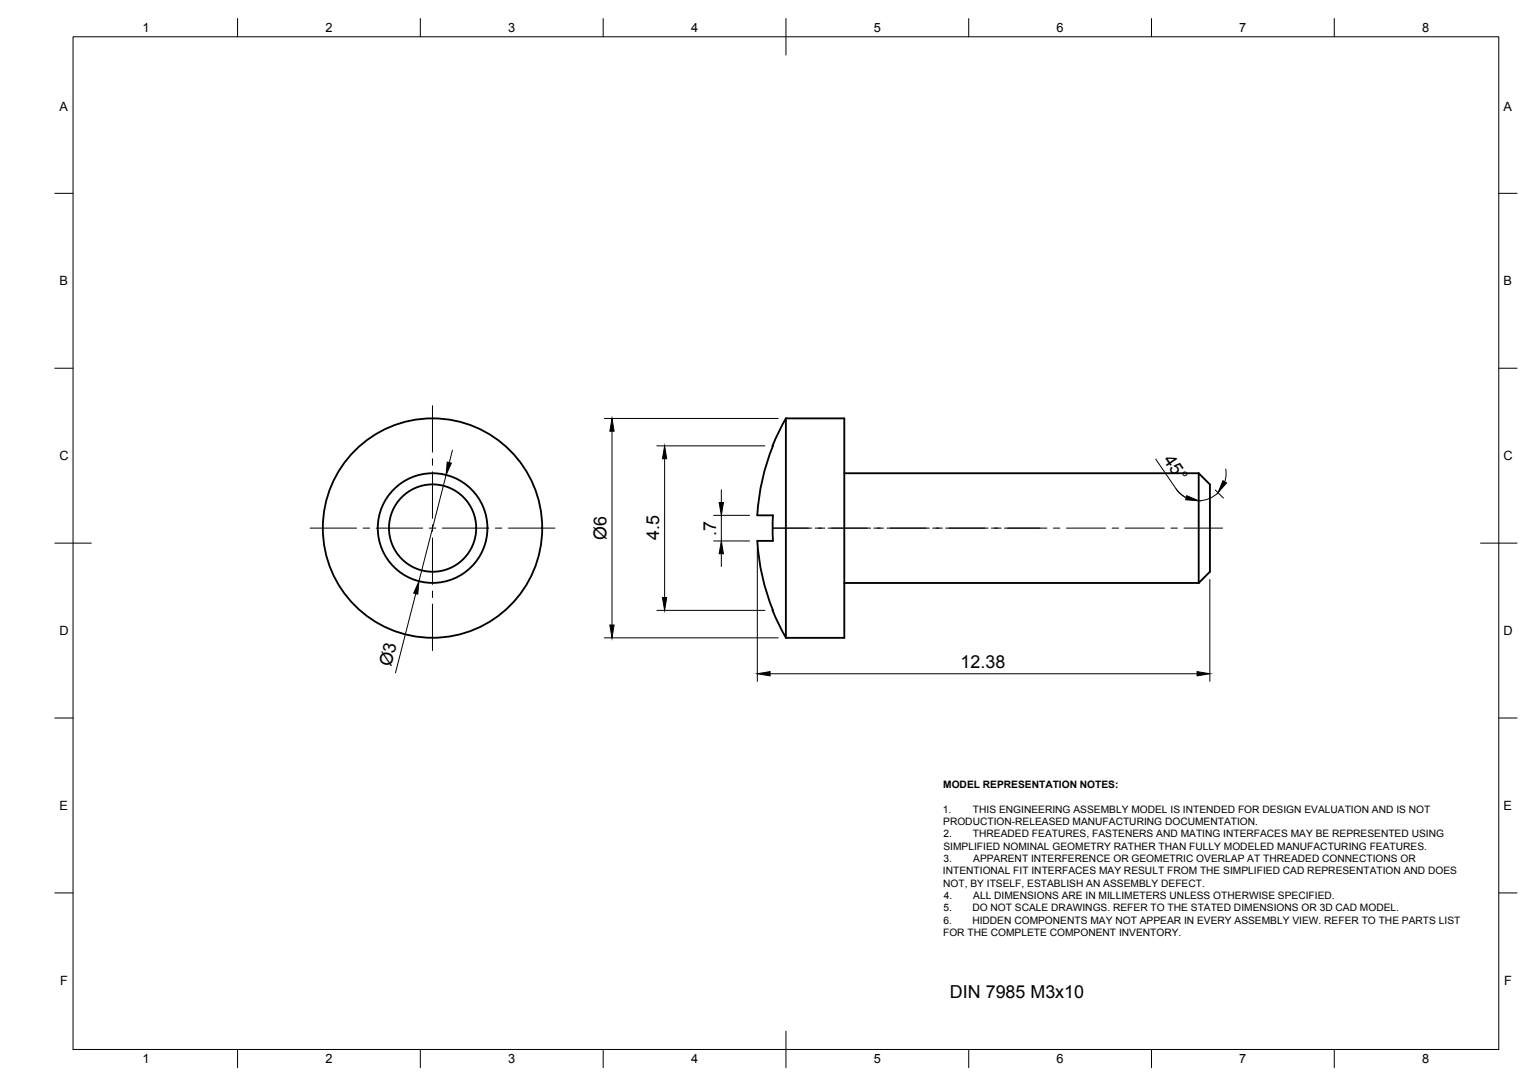
ISO-10303-21;
HEADER;
/* Generated by software containing ST-Developer
 * from STEP Tools, Inc. (www.steptools.com) 
 */

FILE_DESCRIPTION(
/* description */ ('STEP AP214'),
/* implementation_level */ '2;1');

FILE_NAME(
/* name */ 'DIN 7985 M3x10.step',
/* time_stamp */ '2026-10-07T12:18:07-07:00',
/* author */ (''),
/* organization */ (''),
/* preprocessor_version */ 'ST-DEVELOPER v20.2',
/* originating_system */ 'Autodesk Translation Framework v15.15.0.0',
/* authorisation */ '');

FILE_SCHEMA (('AUTOMOTIVE_DESIGN { 1 0 10303 214 3 1 1 }'));
ENDSEC;

DATA;
#10=MECHANICAL_DESIGN_GEOMETRIC_PRESENTATION_REPRESENTATION('',(#127),#62974);
#82=SPHERICAL_SURFACE('',#16177,6.);
#103=SHAPE_REPRESENTATION_RELATIONSHIP('SRR','None',#63026,#115);
#115=ADVANCED_BREP_SHAPE_REPRESENTATION('',(#139),#62967);
#127=STYLED_ITEM('',(#63090),#139);
#139=MANIFOLD_SOLID_BREP('Body1',#15197);
#232=FACE_BOUND('',#5073,.T.);
#233=FACE_BOUND('',#5078,.T.);
#574=PLANE('',#16199);
#575=PLANE('',#16200);
#576=PLANE('',#16201);
#577=PLANE('',#16202);
#578=PLANE('',#16203);
#579=PLANE('',#16204);
#580=PLANE('',#16205);
#581=PLANE('',#16206);
#582=PLANE('',#16207);
#583=PLANE('',#16208);
#584=PLANE('',#16209);
#585=PLANE('',#16210);
#586=PLANE('',#16211);
#587=PLANE('',#16212);
#588=PLANE('',#16213);
#1042=CONICAL_SURFACE('',#16191,1.1935,0.785398163397446);
#1776=LINE('',#44469,#2969);
#1777=LINE('',#44474,#2970);
#1778=LINE('',#44479,#2971);
#1779=LINE('',#44483,#2972);
#1780=LINE('',#44485,#2973);
#1781=LINE('',#44486,#2974);
#1782=LINE('',#44489,#2975);
#1783=LINE('',#44490,#2976);
#1784=LINE('',#44493,#2977);
#1785=LINE('',#44494,#2978);
#1786=LINE('',#44497,#2979);
#1787=LINE('',#44498,#2980);
#1788=LINE('',#44501,#2981);
#1789=LINE('',#44502,#2982);
#1790=LINE('',#44505,#2983);
#1791=LINE('',#44506,#2984);
#1792=LINE('',#44509,#2985);
#1793=LINE('',#44510,#2986);
#1794=LINE('',#44513,#2987);
#1795=LINE('',#44514,#2988);
#1796=LINE('',#44517,#2989);
#1797=LINE('',#44518,#2990);
#1798=LINE('',#44521,#2991);
#1799=LINE('',#44522,#2992);
#1800=LINE('',#44525,#2993);
#1801=LINE('',#44526,#2994);
#1802=LINE('',#44528,#2995);
#2969=VECTOR('',#19387,1.1935);
#2970=VECTOR('',#19394,3.);
#2971=VECTOR('',#19401,1.5);
#2972=VECTOR('',#19406,1000.);
#2973=VECTOR('',#19407,1000.);
#2974=VECTOR('',#19408,1000.);
#2975=VECTOR('',#19411,1000.);
#2976=VECTOR('',#19412,1000.);
#2977=VECTOR('',#19415,1000.);
#2978=VECTOR('',#19416,1000.);
#2979=VECTOR('',#19419,1000.);
#2980=VECTOR('',#19420,1000.);
#2981=VECTOR('',#19423,1000.);
#2982=VECTOR('',#19424,1000.);
#2983=VECTOR('',#19427,1000.);
#2984=VECTOR('',#19428,1000.);
#2985=VECTOR('',#19431,1000.);
#2986=VECTOR('',#19432,1000.);
#2987=VECTOR('',#19435,1000.);
#2988=VECTOR('',#19436,1000.);
#2989=VECTOR('',#19439,1000.);
#2990=VECTOR('',#19440,1000.);
#2991=VECTOR('',#19443,1000.);
#2992=VECTOR('',#19444,1000.);
#2993=VECTOR('',#19447,1000.);
#2994=VECTOR('',#19448,1000.);
#2995=VECTOR('',#19451,1000.);
#3545=CYLINDRICAL_SURFACE('',#16195,3.);
#3546=CYLINDRICAL_SURFACE('',#16197,1.5);
#4167=FACE_OUTER_BOUND('',#5072,.T.);
#4168=FACE_OUTER_BOUND('',#5074,.T.);
#4169=FACE_OUTER_BOUND('',#5075,.T.);
#4170=FACE_OUTER_BOUND('',#5076,.T.);
#4171=FACE_OUTER_BOUND('',#5077,.T.);
#4172=FACE_OUTER_BOUND('',#5079,.T.);
#4173=FACE_OUTER_BOUND('',#5080,.T.);
#4174=FACE_OUTER_BOUND('',#5081,.T.);
#4175=FACE_OUTER_BOUND('',#5082,.T.);
#4176=FACE_OUTER_BOUND('',#5083,.T.);
#4177=FACE_OUTER_BOUND('',#5084,.T.);
#4178=FACE_OUTER_BOUND('',#5085,.T.);
#4179=FACE_OUTER_BOUND('',#5086,.T.);
#4180=FACE_OUTER_BOUND('',#5087,.T.);
#4181=FACE_OUTER_BOUND('',#5088,.T.);
#4182=FACE_OUTER_BOUND('',#5089,.T.);
#4183=FACE_OUTER_BOUND('',#5090,.T.);
#4184=FACE_OUTER_BOUND('',#5091,.T.);
#4185=FACE_OUTER_BOUND('',#5092,.T.);
#5072=EDGE_LOOP('',(#12237));
#5073=EDGE_LOOP('',(#12238,#12239,#12240,#12241,#12242,#12243,#12244,#12245,
#12246,#12247,#12248,#12249));
#5074=EDGE_LOOP('',(#12250,#12251,#12252,#12253,#12254));
#5075=EDGE_LOOP('',(#12255,#12256,#12257,#12258));
#5076=EDGE_LOOP('',(#12259,#12260,#12261,#12262,#12263));
#5077=EDGE_LOOP('',(#12264));
#5078=EDGE_LOOP('',(#12265));
#5079=EDGE_LOOP('',(#12266,#12267,#12268,#12269));
#5080=EDGE_LOOP('',(#12270,#12271,#12272,#12273));
#5081=EDGE_LOOP('',(#12274,#12275,#12276,#12277));
#5082=EDGE_LOOP('',(#12278,#12279,#12280,#12281));
#5083=EDGE_LOOP('',(#12282,#12283,#12284,#12285));
#5084=EDGE_LOOP('',(#12286,#12287,#12288,#12289));
#5085=EDGE_LOOP('',(#12290,#12291,#12292,#12293));
#5086=EDGE_LOOP('',(#12294,#12295,#12296,#12297));
#5087=EDGE_LOOP('',(#12298,#12299,#12300,#12301));
#5088=EDGE_LOOP('',(#12302,#12303,#12304,#12305));
#5089=EDGE_LOOP('',(#12306,#12307,#12308,#12309));
#5090=EDGE_LOOP('',(#12310,#12311,#12312,#12313));
#5091=EDGE_LOOP('',(#12314,#12315,#12316,#12317,#12318,#12319,#12320,#12321,
#12322,#12323,#12324,#12325));
#5092=EDGE_LOOP('',(#12326));
#5854=CIRCLE('',#16178,3.);
#5855=CIRCLE('',#16179,5.56214886532177);
#5856=CIRCLE('',#16180,5.9897829676876);
#5857=CIRCLE('',#16181,5.9897829676876);
#5858=CIRCLE('',#16182,5.5621488653218);
#5859=CIRCLE('',#16183,5.98978296768761);
#5860=CIRCLE('',#16184,5.9897829676876);
#5861=CIRCLE('',#16185,5.56214886532182);
#5862=CIRCLE('',#16186,5.9897829676876);
#5863=CIRCLE('',#16187,5.98978296768761);
#5864=CIRCLE('',#16188,5.5621488653218);
#5865=CIRCLE('',#16189,5.9897829676876);
#5866=CIRCLE('',#16190,5.9897829676876);
#5867=CIRCLE('',#16192,1.5);
#5868=CIRCLE('',#16193,1.1935);
#5869=CIRCLE('',#16194,1.5);
#5870=CIRCLE('',#16196,3.);
#5871=CIRCLE('',#16198,1.5);
#6980=VERTEX_POINT('',#44438);
#6981=VERTEX_POINT('',#44440);
#6982=VERTEX_POINT('',#44441);
#6983=VERTEX_POINT('',#44443);
#6984=VERTEX_POINT('',#44445);
#6985=VERTEX_POINT('',#44447);
#6986=VERTEX_POINT('',#44449);
#6987=VERTEX_POINT('',#44451);
#6988=VERTEX_POINT('',#44453);
#6989=VERTEX_POINT('',#44455);
#6990=VERTEX_POINT('',#44457);
#6991=VERTEX_POINT('',#44459);
#6992=VERTEX_POINT('',#44461);
#6993=VERTEX_POINT('',#44465);
#6994=VERTEX_POINT('',#44466);
#6995=VERTEX_POINT('',#44468);
#6996=VERTEX_POINT('',#44473);
#6997=VERTEX_POINT('',#44477);
#6998=VERTEX_POINT('',#44482);
#6999=VERTEX_POINT('',#44484);
#7000=VERTEX_POINT('',#44488);
#7001=VERTEX_POINT('',#44492);
#7002=VERTEX_POINT('',#44496);
#7003=VERTEX_POINT('',#44500);
#7004=VERTEX_POINT('',#44504);
#7005=VERTEX_POINT('',#44508);
#7006=VERTEX_POINT('',#44512);
#7007=VERTEX_POINT('',#44516);
#7008=VERTEX_POINT('',#44520);
#7009=VERTEX_POINT('',#44524);
#8825=EDGE_CURVE('',#6980,#6980,#5854,.T.);
#8826=EDGE_CURVE('',#6981,#6982,#5855,.T.);
#8827=EDGE_CURVE('',#6982,#6983,#5856,.T.);
#8828=EDGE_CURVE('',#6983,#6984,#5857,.T.);
#8829=EDGE_CURVE('',#6984,#6985,#5858,.T.);
#8830=EDGE_CURVE('',#6985,#6986,#5859,.T.);
#8831=EDGE_CURVE('',#6986,#6987,#5860,.T.);
#8832=EDGE_CURVE('',#6987,#6988,#5861,.T.);
#8833=EDGE_CURVE('',#6988,#6989,#5862,.T.);
#8834=EDGE_CURVE('',#6989,#6990,#5863,.T.);
#8835=EDGE_CURVE('',#6990,#6991,#5864,.T.);
#8836=EDGE_CURVE('',#6991,#6992,#5865,.T.);
#8837=EDGE_CURVE('',#6992,#6981,#5866,.T.);
#8838=EDGE_CURVE('',#6993,#6994,#5867,.T.);
#8839=EDGE_CURVE('',#6994,#6995,#1776,.T.);
#8840=EDGE_CURVE('',#6995,#6995,#5868,.T.);
#8841=EDGE_CURVE('',#6994,#6993,#5869,.T.);
#8842=EDGE_CURVE('',#6980,#6996,#1777,.T.);
#8843=EDGE_CURVE('',#6996,#6996,#5870,.T.);
#8844=EDGE_CURVE('',#6997,#6997,#5871,.T.);
#8845=EDGE_CURVE('',#6997,#6993,#1778,.T.);
#8846=EDGE_CURVE('',#6998,#6991,#1779,.T.);
#8847=EDGE_CURVE('',#6998,#6999,#1780,.T.);
#8848=EDGE_CURVE('',#6999,#6992,#1781,.T.);
#8849=EDGE_CURVE('',#6999,#7000,#1782,.T.);
#8850=EDGE_CURVE('',#7000,#6981,#1783,.T.);
#8851=EDGE_CURVE('',#7000,#7001,#1784,.T.);
#8852=EDGE_CURVE('',#7001,#6982,#1785,.T.);
#8853=EDGE_CURVE('',#7001,#7002,#1786,.T.);
#8854=EDGE_CURVE('',#7002,#6983,#1787,.T.);
#8855=EDGE_CURVE('',#7002,#7003,#1788,.T.);
#8856=EDGE_CURVE('',#7003,#6984,#1789,.T.);
#8857=EDGE_CURVE('',#7003,#7004,#1790,.T.);
#8858=EDGE_CURVE('',#7004,#6985,#1791,.T.);
#8859=EDGE_CURVE('',#7005,#6990,#1792,.T.);
#8860=EDGE_CURVE('',#7005,#6998,#1793,.T.);
#8861=EDGE_CURVE('',#7006,#6989,#1794,.T.);
#8862=EDGE_CURVE('',#7006,#7005,#1795,.T.);
#8863=EDGE_CURVE('',#7004,#7007,#1796,.T.);
#8864=EDGE_CURVE('',#7007,#6986,#1797,.T.);
#8865=EDGE_CURVE('',#7007,#7008,#1798,.T.);
#8866=EDGE_CURVE('',#7008,#6987,#1799,.T.);
#8867=EDGE_CURVE('',#7009,#6988,#1800,.T.);
#8868=EDGE_CURVE('',#7009,#7006,#1801,.T.);
#8869=EDGE_CURVE('',#7008,#7009,#1802,.T.);
#12237=ORIENTED_EDGE('',*,*,#8825,.F.);
#12238=ORIENTED_EDGE('',*,*,#8826,.T.);
#12239=ORIENTED_EDGE('',*,*,#8827,.T.);
#12240=ORIENTED_EDGE('',*,*,#8828,.T.);
#12241=ORIENTED_EDGE('',*,*,#8829,.T.);
#12242=ORIENTED_EDGE('',*,*,#8830,.T.);
#12243=ORIENTED_EDGE('',*,*,#8831,.T.);
#12244=ORIENTED_EDGE('',*,*,#8832,.T.);
#12245=ORIENTED_EDGE('',*,*,#8833,.T.);
#12246=ORIENTED_EDGE('',*,*,#8834,.T.);
#12247=ORIENTED_EDGE('',*,*,#8835,.T.);
#12248=ORIENTED_EDGE('',*,*,#8836,.T.);
#12249=ORIENTED_EDGE('',*,*,#8837,.T.);
#12250=ORIENTED_EDGE('',*,*,#8838,.T.);
#12251=ORIENTED_EDGE('',*,*,#8839,.T.);
#12252=ORIENTED_EDGE('',*,*,#8840,.F.);
#12253=ORIENTED_EDGE('',*,*,#8839,.F.);
#12254=ORIENTED_EDGE('',*,*,#8841,.T.);
#12255=ORIENTED_EDGE('',*,*,#8825,.T.);
#12256=ORIENTED_EDGE('',*,*,#8842,.T.);
#12257=ORIENTED_EDGE('',*,*,#8843,.F.);
#12258=ORIENTED_EDGE('',*,*,#8842,.F.);
#12259=ORIENTED_EDGE('',*,*,#8844,.T.);
#12260=ORIENTED_EDGE('',*,*,#8845,.T.);
#12261=ORIENTED_EDGE('',*,*,#8841,.F.);
#12262=ORIENTED_EDGE('',*,*,#8838,.F.);
#12263=ORIENTED_EDGE('',*,*,#8845,.F.);
#12264=ORIENTED_EDGE('',*,*,#8843,.T.);
#12265=ORIENTED_EDGE('',*,*,#8844,.F.);
#12266=ORIENTED_EDGE('',*,*,#8846,.F.);
#12267=ORIENTED_EDGE('',*,*,#8847,.T.);
#12268=ORIENTED_EDGE('',*,*,#8848,.T.);
#12269=ORIENTED_EDGE('',*,*,#8836,.F.);
#12270=ORIENTED_EDGE('',*,*,#8848,.F.);
#12271=ORIENTED_EDGE('',*,*,#8849,.T.);
#12272=ORIENTED_EDGE('',*,*,#8850,.T.);
#12273=ORIENTED_EDGE('',*,*,#8837,.F.);
#12274=ORIENTED_EDGE('',*,*,#8850,.F.);
#12275=ORIENTED_EDGE('',*,*,#8851,.T.);
#12276=ORIENTED_EDGE('',*,*,#8852,.T.);
#12277=ORIENTED_EDGE('',*,*,#8826,.F.);
#12278=ORIENTED_EDGE('',*,*,#8852,.F.);
#12279=ORIENTED_EDGE('',*,*,#8853,.T.);
#12280=ORIENTED_EDGE('',*,*,#8854,.T.);
#12281=ORIENTED_EDGE('',*,*,#8827,.F.);
#12282=ORIENTED_EDGE('',*,*,#8854,.F.);
#12283=ORIENTED_EDGE('',*,*,#8855,.T.);
#12284=ORIENTED_EDGE('',*,*,#8856,.T.);
#12285=ORIENTED_EDGE('',*,*,#8828,.F.);
#12286=ORIENTED_EDGE('',*,*,#8856,.F.);
#12287=ORIENTED_EDGE('',*,*,#8857,.T.);
#12288=ORIENTED_EDGE('',*,*,#8858,.T.);
#12289=ORIENTED_EDGE('',*,*,#8829,.F.);
#12290=ORIENTED_EDGE('',*,*,#8859,.F.);
#12291=ORIENTED_EDGE('',*,*,#8860,.T.);
#12292=ORIENTED_EDGE('',*,*,#8846,.T.);
#12293=ORIENTED_EDGE('',*,*,#8835,.F.);
#12294=ORIENTED_EDGE('',*,*,#8861,.F.);
#12295=ORIENTED_EDGE('',*,*,#8862,.T.);
#12296=ORIENTED_EDGE('',*,*,#8859,.T.);
#12297=ORIENTED_EDGE('',*,*,#8834,.F.);
#12298=ORIENTED_EDGE('',*,*,#8858,.F.);
#12299=ORIENTED_EDGE('',*,*,#8863,.T.);
#12300=ORIENTED_EDGE('',*,*,#8864,.T.);
#12301=ORIENTED_EDGE('',*,*,#8830,.F.);
#12302=ORIENTED_EDGE('',*,*,#8864,.F.);
#12303=ORIENTED_EDGE('',*,*,#8865,.T.);
#12304=ORIENTED_EDGE('',*,*,#8866,.T.);
#12305=ORIENTED_EDGE('',*,*,#8831,.F.);
#12306=ORIENTED_EDGE('',*,*,#8867,.F.);
#12307=ORIENTED_EDGE('',*,*,#8868,.T.);
#12308=ORIENTED_EDGE('',*,*,#8861,.T.);
#12309=ORIENTED_EDGE('',*,*,#8833,.F.);
#12310=ORIENTED_EDGE('',*,*,#8866,.F.);
#12311=ORIENTED_EDGE('',*,*,#8869,.T.);
#12312=ORIENTED_EDGE('',*,*,#8867,.T.);
#12313=ORIENTED_EDGE('',*,*,#8832,.F.);
#12314=ORIENTED_EDGE('',*,*,#8869,.F.);
#12315=ORIENTED_EDGE('',*,*,#8865,.F.);
#12316=ORIENTED_EDGE('',*,*,#8863,.F.);
#12317=ORIENTED_EDGE('',*,*,#8857,.F.);
#12318=ORIENTED_EDGE('',*,*,#8855,.F.);
#12319=ORIENTED_EDGE('',*,*,#8853,.F.);
#12320=ORIENTED_EDGE('',*,*,#8851,.F.);
#12321=ORIENTED_EDGE('',*,*,#8849,.F.);
#12322=ORIENTED_EDGE('',*,*,#8847,.F.);
#12323=ORIENTED_EDGE('',*,*,#8860,.F.);
#12324=ORIENTED_EDGE('',*,*,#8862,.F.);
#12325=ORIENTED_EDGE('',*,*,#8868,.F.);
#12326=ORIENTED_EDGE('',*,*,#8840,.T.);
#14802=ADVANCED_FACE('',(#4167,#232),#82,.T.);
#14803=ADVANCED_FACE('',(#4168),#1042,.T.);
#14804=ADVANCED_FACE('',(#4169),#3545,.T.);
#14805=ADVANCED_FACE('',(#4170),#3546,.T.);
#14806=ADVANCED_FACE('',(#4171,#233),#574,.T.);
#14807=ADVANCED_FACE('',(#4172),#575,.T.);
#14808=ADVANCED_FACE('',(#4173),#576,.T.);
#14809=ADVANCED_FACE('',(#4174),#577,.T.);
#14810=ADVANCED_FACE('',(#4175),#578,.T.);
#14811=ADVANCED_FACE('',(#4176),#579,.T.);
#14812=ADVANCED_FACE('',(#4177),#580,.T.);
#14813=ADVANCED_FACE('',(#4178),#581,.T.);
#14814=ADVANCED_FACE('',(#4179),#582,.T.);
#14815=ADVANCED_FACE('',(#4180),#583,.T.);
#14816=ADVANCED_FACE('',(#4181),#584,.T.);
#14817=ADVANCED_FACE('',(#4182),#585,.T.);
#14818=ADVANCED_FACE('',(#4183),#586,.T.);
#14819=ADVANCED_FACE('',(#4184),#587,.F.);
#14820=ADVANCED_FACE('',(#4185),#588,.T.);
#15197=CLOSED_SHELL('',(#14802,#14803,#14804,#14805,#14806,#14807,#14808,
#14809,#14810,#14811,#14812,#14813,#14814,#14815,#14816,#14817,#14818,#14819,
#14820));
#16176=AXIS2_PLACEMENT_3D('',#44436,#19353,#19354);
#16177=AXIS2_PLACEMENT_3D('',#44437,#19355,#19356);
#16178=AXIS2_PLACEMENT_3D('',#44439,#19357,#19358);
#16179=AXIS2_PLACEMENT_3D('',#44442,#19359,#19360);
#16180=AXIS2_PLACEMENT_3D('',#44444,#19361,#19362);
#16181=AXIS2_PLACEMENT_3D('',#44446,#19363,#19364);
#16182=AXIS2_PLACEMENT_3D('',#44448,#19365,#19366);
#16183=AXIS2_PLACEMENT_3D('',#44450,#19367,#19368);
#16184=AXIS2_PLACEMENT_3D('',#44452,#19369,#19370);
#16185=AXIS2_PLACEMENT_3D('',#44454,#19371,#19372);
#16186=AXIS2_PLACEMENT_3D('',#44456,#19373,#19374);
#16187=AXIS2_PLACEMENT_3D('',#44458,#19375,#19376);
#16188=AXIS2_PLACEMENT_3D('',#44460,#19377,#19378);
#16189=AXIS2_PLACEMENT_3D('',#44462,#19379,#19380);
#16190=AXIS2_PLACEMENT_3D('',#44463,#19381,#19382);
#16191=AXIS2_PLACEMENT_3D('',#44464,#19383,#19384);
#16192=AXIS2_PLACEMENT_3D('',#44467,#19385,#19386);
#16193=AXIS2_PLACEMENT_3D('',#44470,#19388,#19389);
#16194=AXIS2_PLACEMENT_3D('',#44471,#19390,#19391);
#16195=AXIS2_PLACEMENT_3D('',#44472,#19392,#19393);
#16196=AXIS2_PLACEMENT_3D('',#44475,#19395,#19396);
#16197=AXIS2_PLACEMENT_3D('',#44476,#19397,#19398);
#16198=AXIS2_PLACEMENT_3D('',#44478,#19399,#19400);
#16199=AXIS2_PLACEMENT_3D('',#44480,#19402,#19403);
#16200=AXIS2_PLACEMENT_3D('',#44481,#19404,#19405);
#16201=AXIS2_PLACEMENT_3D('',#44487,#19409,#19410);
#16202=AXIS2_PLACEMENT_3D('',#44491,#19413,#19414);
#16203=AXIS2_PLACEMENT_3D('',#44495,#19417,#19418);
#16204=AXIS2_PLACEMENT_3D('',#44499,#19421,#19422);
#16205=AXIS2_PLACEMENT_3D('',#44503,#19425,#19426);
#16206=AXIS2_PLACEMENT_3D('',#44507,#19429,#19430);
#16207=AXIS2_PLACEMENT_3D('',#44511,#19433,#19434);
#16208=AXIS2_PLACEMENT_3D('',#44515,#19437,#19438);
#16209=AXIS2_PLACEMENT_3D('',#44519,#19441,#19442);
#16210=AXIS2_PLACEMENT_3D('',#44523,#19445,#19446);
#16211=AXIS2_PLACEMENT_3D('',#44527,#19449,#19450);
#16212=AXIS2_PLACEMENT_3D('',#44529,#19452,#19453);
#16213=AXIS2_PLACEMENT_3D('',#44530,#19454,#19455);
#19353=DIRECTION('axis',(0.,0.,1.));
#19354=DIRECTION('refdir',(1.,0.,0.));
#19355=DIRECTION('center_axis',(1.1842378929335E-15,1.1842378929335E-15,
-1.));
#19356=DIRECTION('ref_axis',(1.1842378929335E-15,1.,1.03620815631681E-15));
#19357=DIRECTION('center_axis',(-1.,1.E-15,-1.E-15));
#19358=DIRECTION('ref_axis',(-1.E-15,-1.15648231731787E-15,1.));
#19359=DIRECTION('center_axis',(1.E-15,1.,1.E-15));
#19360=DIRECTION('ref_axis',(-1.247520350843E-15,-9.99999999999999E-16,
1.));
#19361=DIRECTION('center_axis',(1.E-15,1.E-15,-1.));
#19362=DIRECTION('ref_axis',(1.15845497931055E-15,1.,1.E-15));
#19363=DIRECTION('center_axis',(1.E-15,1.,1.E-15));
#19364=DIRECTION('ref_axis',(-1.15845497931055E-15,-9.99999999999999E-16,
1.));
#19365=DIRECTION('center_axis',(1.E-15,1.E-15,-1.));
#19366=DIRECTION('ref_axis',(1.247520350843E-15,1.,1.E-15));
#19367=DIRECTION('center_axis',(-1.E-15,-1.,-1.E-15));
#19368=DIRECTION('ref_axis',(1.15845497931055E-15,9.99999999999999E-16,
-1.));
#19369=DIRECTION('center_axis',(1.E-15,1.E-15,-1.));
#19370=DIRECTION('ref_axis',(1.15845497931055E-15,1.,1.E-15));
#19371=DIRECTION('center_axis',(-1.E-15,-1.,-1.E-15));
#19372=DIRECTION('ref_axis',(1.24752035084299E-15,9.99999999999999E-16,
-1.));
#19373=DIRECTION('center_axis',(-1.E-15,-1.E-15,1.));
#19374=DIRECTION('ref_axis',(-1.15845497931055E-15,-1.,-1.E-15));
#19375=DIRECTION('center_axis',(-1.E-15,-1.,-1.E-15));
#19376=DIRECTION('ref_axis',(1.15845497931055E-15,9.99999999999999E-16,
-1.));
#19377=DIRECTION('center_axis',(-1.E-15,-1.E-15,1.));
#19378=DIRECTION('ref_axis',(-1.247520350843E-15,-1.,-1.E-15));
#19379=DIRECTION('center_axis',(1.E-15,1.,1.E-15));
#19380=DIRECTION('ref_axis',(-1.15845497931055E-15,-9.99999999999999E-16,
1.));
#19381=DIRECTION('center_axis',(-1.E-15,-1.E-15,1.));
#19382=DIRECTION('ref_axis',(-1.15845497931055E-15,-1.,-1.E-15));
#19383=DIRECTION('center_axis',(1.,-1.E-15,1.E-15));
#19384=DIRECTION('ref_axis',(1.E-15,-1.E-30,-1.));
#19385=DIRECTION('center_axis',(-1.,1.E-15,-1.E-15));
#19386=DIRECTION('ref_axis',(-1.E-15,1.E-30,1.));
#19387=DIRECTION('',(-0.707106781186548,7.93702386810097E-16,-0.707106781186547));
#19388=DIRECTION('center_axis',(-1.,1.E-15,-1.E-15));
#19389=DIRECTION('ref_axis',(-1.E-15,1.E-30,1.));
#19390=DIRECTION('center_axis',(-1.,1.E-15,-1.E-15));
#19391=DIRECTION('ref_axis',(-1.E-15,1.E-30,1.));
#19392=DIRECTION('center_axis',(1.,-1.E-15,1.E-15));
#19393=DIRECTION('ref_axis',(-1.E-15,-1.15648231731787E-15,1.));
#19394=DIRECTION('',(-1.,1.E-15,-1.E-15));
#19395=DIRECTION('center_axis',(-1.,1.E-15,-1.E-15));
#19396=DIRECTION('ref_axis',(-1.E-15,-1.15648231731787E-15,1.));
#19397=DIRECTION('center_axis',(1.,-1.E-15,1.E-15));
#19398=DIRECTION('ref_axis',(-1.E-15,1.E-30,1.));
#19399=DIRECTION('center_axis',(-1.,1.E-15,-1.E-15));
#19400=DIRECTION('ref_axis',(-1.E-15,1.E-30,1.));
#19401=DIRECTION('',(-1.,1.E-15,-1.E-15));
#19402=DIRECTION('center_axis',(-1.,1.E-15,-1.E-15));
#19403=DIRECTION('ref_axis',(1.E-15,1.,1.E-15));
#19404=DIRECTION('center_axis',(-1.E-15,-1.,-1.E-15));
#19405=DIRECTION('ref_axis',(-1.E-15,-1.E-15,1.));
#19406=DIRECTION('',(1.,-1.E-15,1.E-15));
#19407=DIRECTION('',(1.E-15,1.E-15,-1.));
#19408=DIRECTION('',(1.,-1.E-15,1.E-15));
#19409=DIRECTION('center_axis',(1.E-15,1.E-15,-1.));
#19410=DIRECTION('ref_axis',(1.,-1.E-15,1.E-15));
#19411=DIRECTION('',(1.E-15,1.,1.E-15));
#19412=DIRECTION('',(1.,-1.E-15,1.E-15));
#19413=DIRECTION('center_axis',(-1.E-15,-1.,-1.E-15));
#19414=DIRECTION('ref_axis',(-1.E-15,-1.E-15,1.));
#19415=DIRECTION('',(1.E-15,1.E-15,-1.));
#19416=DIRECTION('',(1.,-1.E-15,1.E-15));
#19417=DIRECTION('center_axis',(-1.E-15,-9.99999999999999E-16,1.));
#19418=DIRECTION('ref_axis',(1.E-15,1.,1.E-15));
#19419=DIRECTION('',(-1.E-15,-1.,-1.E-15));
#19420=DIRECTION('',(1.,-1.E-15,1.E-15));
#19421=DIRECTION('center_axis',(-1.E-15,-1.,-1.E-15));
#19422=DIRECTION('ref_axis',(-1.E-15,-1.E-15,1.));
#19423=DIRECTION('',(1.E-15,1.E-15,-1.));
#19424=DIRECTION('',(1.,-1.E-15,1.E-15));
#19425=DIRECTION('center_axis',(-1.E-15,-9.99999999999999E-16,1.));
#19426=DIRECTION('ref_axis',(1.E-15,1.,1.E-15));
#19427=DIRECTION('',(-1.E-15,-1.,-1.E-15));
#19428=DIRECTION('',(1.,-1.E-15,1.E-15));
#19429=DIRECTION('center_axis',(1.E-15,1.E-15,-1.));
#19430=DIRECTION('ref_axis',(1.,-1.E-15,1.E-15));
#19431=DIRECTION('',(1.,-1.E-15,1.E-15));
#19432=DIRECTION('',(1.E-15,1.,1.E-15));
#19433=DIRECTION('center_axis',(9.99999999999999E-16,1.,1.E-15));
#19434=DIRECTION('ref_axis',(-1.,1.E-15,-1.E-15));
#19435=DIRECTION('',(1.,-1.E-15,1.E-15));
#19436=DIRECTION('',(-1.E-15,-1.E-15,1.));
#19437=DIRECTION('center_axis',(9.99999999999999E-16,1.,1.E-15));
#19438=DIRECTION('ref_axis',(-1.,1.E-15,-1.E-15));
#19439=DIRECTION('',(-1.E-15,-1.E-15,1.));
#19440=DIRECTION('',(1.,-1.E-15,1.E-15));
#19441=DIRECTION('center_axis',(-1.E-15,-9.99999999999999E-16,1.));
#19442=DIRECTION('ref_axis',(1.E-15,1.,1.E-15));
#19443=DIRECTION('',(-1.E-15,-1.,-1.E-15));
#19444=DIRECTION('',(1.,-1.E-15,1.E-15));
#19445=DIRECTION('center_axis',(1.E-15,1.E-15,-1.));
#19446=DIRECTION('ref_axis',(1.,-1.E-15,1.E-15));
#19447=DIRECTION('',(1.,-1.E-15,1.E-15));
#19448=DIRECTION('',(1.E-15,1.,1.E-15));
#19449=DIRECTION('center_axis',(9.99999999999999E-16,1.,1.E-15));
#19450=DIRECTION('ref_axis',(-1.,1.E-15,-1.E-15));
#19451=DIRECTION('',(-1.E-15,-1.E-15,1.));
#19452=DIRECTION('center_axis',(-1.,1.E-15,-1.E-15));
#19453=DIRECTION('ref_axis',(1.E-15,1.,1.E-15));
#19454=DIRECTION('center_axis',(-1.,1.E-15,-1.E-15));
#19455=DIRECTION('ref_axis',(1.E-15,1.,1.E-15));
#44436=CARTESIAN_POINT('',(0.,0.,0.));
#44437=CARTESIAN_POINT('Origin',(32.2,20.9999992399189,6.));
#44438=CARTESIAN_POINT('',(37.3961524227066,20.999999239919,3.));
#44439=CARTESIAN_POINT('Origin',(37.3961524227066,20.999999239919,6.));
#44440=CARTESIAN_POINT('',(37.7511260119006,23.249999239919,6.35));
#44441=CARTESIAN_POINT('',(37.7511260119006,23.249999239919,5.65));
#44442=CARTESIAN_POINT('Origin',(32.2,23.249999239919,6.));
#44443=CARTESIAN_POINT('',(38.1795484779371,21.349999239919,5.65));
#44444=CARTESIAN_POINT('Origin',(32.2,20.9999992399189,5.65));
#44445=CARTESIAN_POINT('',(37.7511260119007,21.349999239919,3.75));
#44446=CARTESIAN_POINT('Origin',(32.2,21.349999239919,6.));
#44447=CARTESIAN_POINT('',(37.7511260119007,20.649999239919,3.75));
#44448=CARTESIAN_POINT('Origin',(32.2,20.9999992399189,3.75));
#44449=CARTESIAN_POINT('',(38.1795484779371,20.649999239919,5.65));
#44450=CARTESIAN_POINT('Origin',(32.2,20.649999239919,6.));
#44451=CARTESIAN_POINT('',(37.7511260119007,18.749999239919,5.65));
#44452=CARTESIAN_POINT('Origin',(32.2,20.9999992399189,5.65));
#44453=CARTESIAN_POINT('',(37.7511260119007,18.749999239919,6.35));
#44454=CARTESIAN_POINT('Origin',(32.2,18.749999239919,5.99999999999999));
#44455=CARTESIAN_POINT('',(38.1795484779371,20.649999239919,6.35));
#44456=CARTESIAN_POINT('Origin',(32.2,20.9999992399189,6.35));
#44457=CARTESIAN_POINT('',(37.7511260119007,20.649999239919,8.25));
#44458=CARTESIAN_POINT('Origin',(32.2,20.649999239919,6.));
#44459=CARTESIAN_POINT('',(37.7511260119007,21.349999239919,8.25));
#44460=CARTESIAN_POINT('Origin',(32.2,20.9999992399189,8.25));
#44461=CARTESIAN_POINT('',(38.1795484779371,21.349999239919,6.35));
#44462=CARTESIAN_POINT('Origin',(32.2,21.349999239919,6.));
#44463=CARTESIAN_POINT('Origin',(32.2,20.9999992399189,6.35));
#44464=CARTESIAN_POINT('Origin',(25.8,20.999999239919,5.99999999999999));
#44465=CARTESIAN_POINT('',(26.1065,20.999999239919,4.49999999999999));
#44466=CARTESIAN_POINT('',(26.1065,20.999999239919,7.49999999999999));
#44467=CARTESIAN_POINT('Origin',(26.1065,20.999999239919,5.99999999999999));
#44468=CARTESIAN_POINT('',(25.8,20.999999239919,7.19349999999999));
#44469=CARTESIAN_POINT('',(25.8,20.999999239919,7.19349999999999));
#44470=CARTESIAN_POINT('Origin',(25.8,20.999999239919,5.99999999999999));
#44471=CARTESIAN_POINT('Origin',(26.1065,20.999999239919,5.99999999999999));
#44472=CARTESIAN_POINT('Origin',(85.8,20.9999992399189,6.00000000000005));
#44473=CARTESIAN_POINT('',(35.8,20.999999239919,3.));
#44474=CARTESIAN_POINT('',(85.8,20.999999239919,3.00000000000005));
#44475=CARTESIAN_POINT('Origin',(35.8,20.999999239919,6.));
#44476=CARTESIAN_POINT('Origin',(85.8,20.9999992399189,6.00000000000005));
#44477=CARTESIAN_POINT('',(35.8,20.999999239919,4.5));
#44478=CARTESIAN_POINT('Origin',(35.8,20.999999239919,6.));
#44479=CARTESIAN_POINT('',(85.8,20.9999992399189,4.50000000000005));
#44480=CARTESIAN_POINT('Origin',(35.8,22.499999239919,6.));
#44481=CARTESIAN_POINT('Origin',(36.4,21.349999239919,8.25));
#44482=CARTESIAN_POINT('',(36.4,21.349999239919,8.25));
#44483=CARTESIAN_POINT('',(36.4,21.349999239919,8.25));
#44484=CARTESIAN_POINT('',(36.4,21.349999239919,6.35));
#44485=CARTESIAN_POINT('',(36.4,21.349999239919,8.25));
#44486=CARTESIAN_POINT('',(36.4,21.349999239919,6.35));
#44487=CARTESIAN_POINT('Origin',(36.4,21.349999239919,6.35));
#44488=CARTESIAN_POINT('',(36.4,23.249999239919,6.35));
#44489=CARTESIAN_POINT('',(36.4,21.349999239919,6.35));
#44490=CARTESIAN_POINT('',(36.4,23.249999239919,6.35));
#44491=CARTESIAN_POINT('Origin',(36.4,23.249999239919,6.35));
#44492=CARTESIAN_POINT('',(36.4,23.249999239919,5.65));
#44493=CARTESIAN_POINT('',(36.4,23.249999239919,6.35));
#44494=CARTESIAN_POINT('',(36.4,23.249999239919,5.65));
#44495=CARTESIAN_POINT('Origin',(36.4,23.249999239919,5.65));
#44496=CARTESIAN_POINT('',(36.4,21.349999239919,5.65));
#44497=CARTESIAN_POINT('',(36.4,23.249999239919,5.65));
#44498=CARTESIAN_POINT('',(36.4,21.349999239919,5.65));
#44499=CARTESIAN_POINT('Origin',(36.4,21.349999239919,5.65));
#44500=CARTESIAN_POINT('',(36.4,21.349999239919,3.75));
#44501=CARTESIAN_POINT('',(36.4,21.349999239919,5.65));
#44502=CARTESIAN_POINT('',(36.4,21.349999239919,3.75));
#44503=CARTESIAN_POINT('Origin',(36.4,21.349999239919,3.75));
#44504=CARTESIAN_POINT('',(36.4,20.649999239919,3.75));
#44505=CARTESIAN_POINT('',(36.4,21.349999239919,3.75));
#44506=CARTESIAN_POINT('',(36.4,20.649999239919,3.75));
#44507=CARTESIAN_POINT('Origin',(36.4,20.649999239919,8.25));
#44508=CARTESIAN_POINT('',(36.4,20.649999239919,8.25));
#44509=CARTESIAN_POINT('',(36.4,20.649999239919,8.25));
#44510=CARTESIAN_POINT('',(36.4,20.649999239919,8.25));
#44511=CARTESIAN_POINT('Origin',(36.4,20.649999239919,6.35));
#44512=CARTESIAN_POINT('',(36.4,20.649999239919,6.35));
#44513=CARTESIAN_POINT('',(36.4,20.649999239919,6.35));
#44514=CARTESIAN_POINT('',(36.4,20.649999239919,6.35));
#44515=CARTESIAN_POINT('Origin',(36.4,20.649999239919,3.75));
#44516=CARTESIAN_POINT('',(36.4,20.649999239919,5.65));
#44517=CARTESIAN_POINT('',(36.4,20.649999239919,3.75));
#44518=CARTESIAN_POINT('',(36.4,20.649999239919,5.65));
#44519=CARTESIAN_POINT('Origin',(36.4,20.649999239919,5.65));
#44520=CARTESIAN_POINT('',(36.4,18.749999239919,5.65));
#44521=CARTESIAN_POINT('',(36.4,20.649999239919,5.65));
#44522=CARTESIAN_POINT('',(36.4,18.749999239919,5.65));
#44523=CARTESIAN_POINT('Origin',(36.4,18.749999239919,6.35));
#44524=CARTESIAN_POINT('',(36.4,18.749999239919,6.35));
#44525=CARTESIAN_POINT('',(36.4,18.749999239919,6.35));
#44526=CARTESIAN_POINT('',(36.4,18.749999239919,6.35));
#44527=CARTESIAN_POINT('Origin',(36.4,18.749999239919,5.65));
#44528=CARTESIAN_POINT('',(36.4,18.749999239919,5.65));
#44529=CARTESIAN_POINT('Origin',(36.4,18.749999239919,6.35));
#44530=CARTESIAN_POINT('Origin',(25.8,20.999999239919,5.99999999999999));
#62953=UNCERTAINTY_MEASURE_WITH_UNIT(LENGTH_MEASURE(0.01),#62975,
'DISTANCE_ACCURACY_VALUE',
'Maximum model space distance between geometric entities at asserted c
onnectivities');
#62960=UNCERTAINTY_MEASURE_WITH_UNIT(LENGTH_MEASURE(0.01),#62975,
'DISTANCE_ACCURACY_VALUE',
'Maximum model space distance between geometric entities at asserted c
onnectivities');
#62967=(
GEOMETRIC_REPRESENTATION_CONTEXT(3)
GLOBAL_UNCERTAINTY_ASSIGNED_CONTEXT((#62953))
GLOBAL_UNIT_ASSIGNED_CONTEXT((#62975,#62977,#62978))
REPRESENTATION_CONTEXT('','3D')
);
#62974=(
GEOMETRIC_REPRESENTATION_CONTEXT(3)
GLOBAL_UNCERTAINTY_ASSIGNED_CONTEXT((#62960))
GLOBAL_UNIT_ASSIGNED_CONTEXT((#62975,#62977,#62978))
REPRESENTATION_CONTEXT('','3D')
);
#62975=(
LENGTH_UNIT()
NAMED_UNIT(*)
SI_UNIT(.MILLI.,.METRE.)
);
#62977=(
NAMED_UNIT(*)
PLANE_ANGLE_UNIT()
SI_UNIT($,.RADIAN.)
);
#62978=(
NAMED_UNIT(*)
SI_UNIT($,.STERADIAN.)
SOLID_ANGLE_UNIT()
);
#62985=SHAPE_DEFINITION_REPRESENTATION(#62998,#63026);
#62998=PRODUCT_DEFINITION_SHAPE('',$,#63040);
#63026=SHAPE_REPRESENTATION('',(#16176),#62967);
#63033=PRODUCT_DEFINITION_CONTEXT('part definition',#63074,'design');
#63040=PRODUCT_DEFINITION('DIN 7985 M3x10','DIN 7985 M3x10',#63053,#63033);
#63053=PRODUCT_DEFINITION_FORMATION('',$,#63082);
#63074=APPLICATION_CONTEXT(
'Core Data for Automotive Mechanical Design Process');
#63075=PRODUCT_CONTEXT('part definition',#63074,'mechanical');
#63082=PRODUCT('DIN 7985 M3x10','DIN 7985 M3x10',$,(#63075));
#63090=PRESENTATION_STYLE_ASSIGNMENT((#63092));
#63092=SURFACE_STYLE_USAGE(.BOTH.,#63094);
#63094=SURFACE_SIDE_STYLE('',(#63096));
#63096=SURFACE_STYLE_FILL_AREA(#63098);
#63098=FILL_AREA_STYLE('Opaque(202,209,238)',(#63100));
#63100=FILL_AREA_STYLE_COLOUR('Opaque(202,209,238)',#63102);
#63102=COLOUR_RGB('Opaque(202,209,238)', 0.66274510, 0.83137255, 0.94901961);
ENDSEC;
END-ISO-10303-21;
